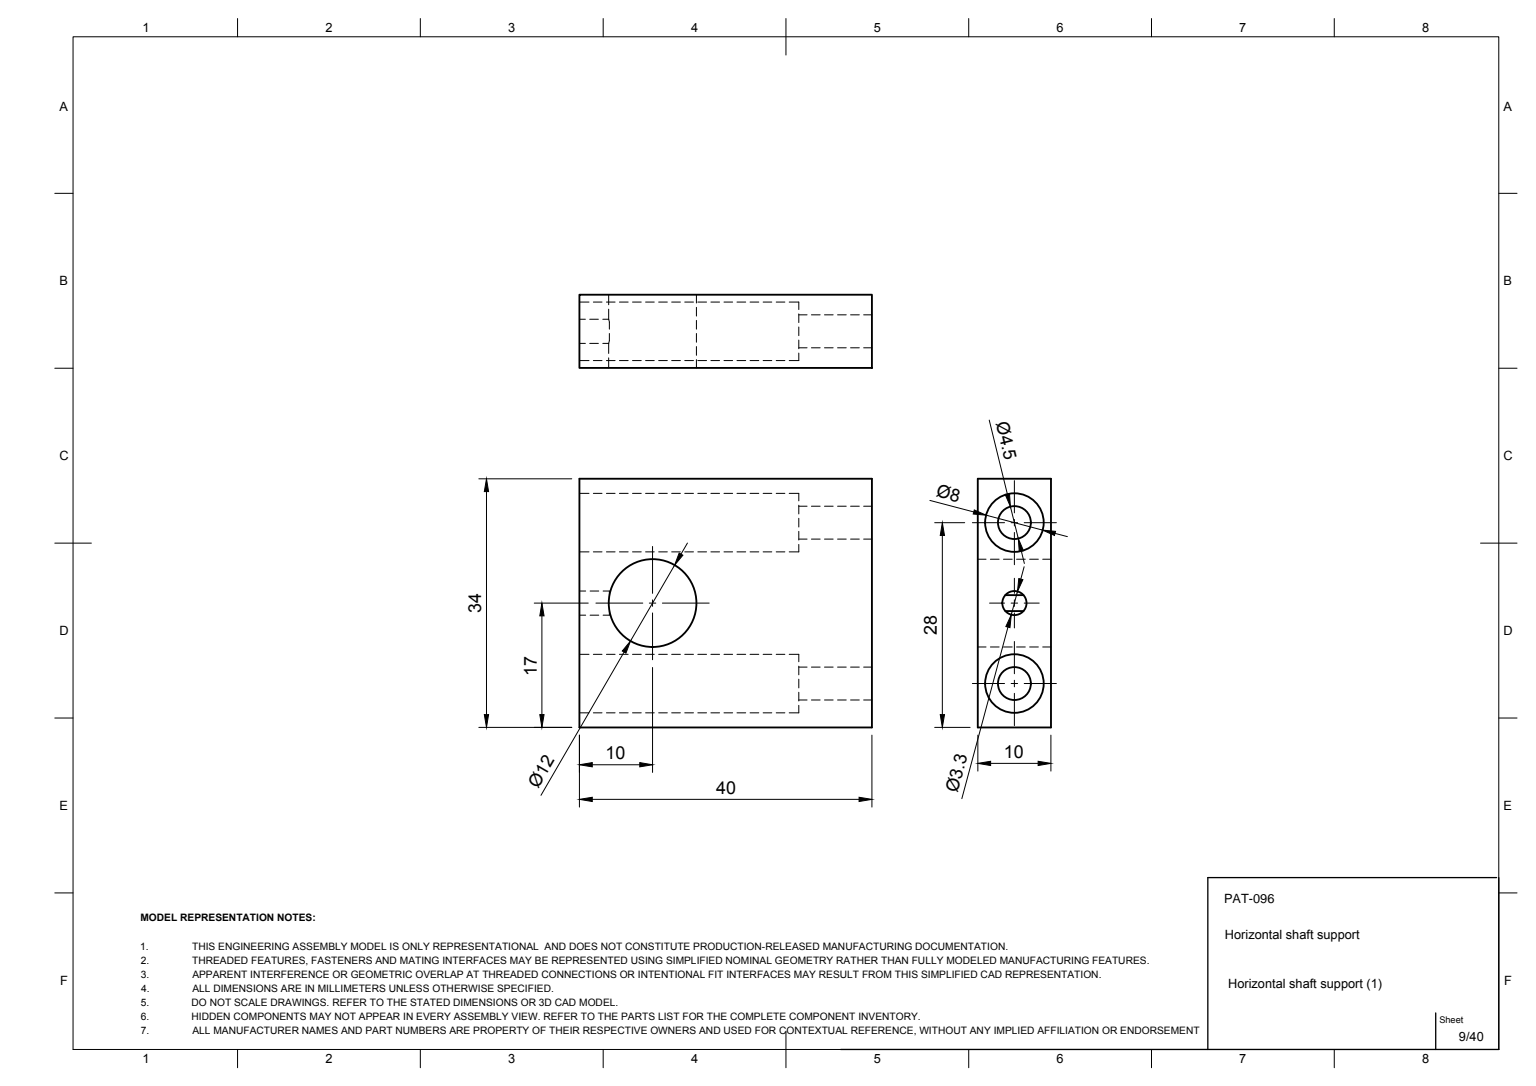
ISO-10303-21;
HEADER;
/* Generated by software containing ST-Developer
 * from STEP Tools, Inc. (www.steptools.com) 
 */

FILE_DESCRIPTION(
/* description */ ('PAT-096'),
/* implementation_level */ '2;1');

FILE_NAME(
/* name */ 'Horizontal shaft support.step',
/* time_stamp */ '2026-10-29T17:03:14-07:00',
/* author */ (''),
/* organization */ (''),
/* preprocessor_version */ 'ST-DEVELOPER v20.2',
/* originating_system */ 'Autodesk Translation Framework v15.17.0.0',
/* authorisation */ '');

FILE_SCHEMA (('AUTOMOTIVE_DESIGN { 1 0 10303 214 3 1 1 }'));
ENDSEC;

DATA;
#10=MECHANICAL_DESIGN_GEOMETRIC_PRESENTATION_REPRESENTATION('',(#416),#10650);
#303=B_SPLINE_CURVE_WITH_KNOTS('',3,(#9562,#9563,#9564,#9565,#9566,#9567),
 .UNSPECIFIED.,.F.,.F.,(4,2,4),(0.635430324955934,0.687528937234029,0.750024497760675),
 .UNSPECIFIED.);
#304=B_SPLINE_CURVE_WITH_KNOTS('',3,(#9571,#9572,#9573,#9574,#9575,#9576),
 .UNSPECIFIED.,.F.,.F.,(4,2,4),(0.250008165920225,0.312503726446871,0.364602338724967),
 .UNSPECIFIED.);
#305=B_SPLINE_CURVE_WITH_KNOTS('',3,(#9577,#9578,#9579,#9580,#9581,#9582),
 .UNSPECIFIED.,.F.,.F.,(4,2,4),(0.135413993115484,0.187512605393579,0.250008165920225),
 .UNSPECIFIED.);
#306=B_SPLINE_CURVE_WITH_KNOTS('',3,(#9583,#9584,#9585,#9586,#9587,#9588),
 .UNSPECIFIED.,.F.,.F.,(4,2,4),(0.750024497760675,0.81252005828732,0.864618670565416),
 .UNSPECIFIED.);
#346=SHAPE_REPRESENTATION_RELATIONSHIP('SRR','None',#10807,#377);
#377=ADVANCED_BREP_SHAPE_REPRESENTATION('',(#454),#10625);
#416=STYLED_ITEM('',(#11064),#454);
#454=MANIFOLD_SOLID_BREP('Body1',#5550);
#532=FACE_BOUND('',#1324,.T.);
#533=FACE_BOUND('',#1327,.T.);
#534=FACE_BOUND('',#1329,.T.);
#535=FACE_BOUND('',#1330,.T.);
#536=FACE_BOUND('',#1331,.T.);
#537=FACE_BOUND('',#1336,.T.);
#538=FACE_BOUND('',#1338,.T.);
#539=FACE_BOUND('',#1340,.T.);
#540=FACE_BOUND('',#1341,.T.);
#667=PLANE('',#6226);
#668=PLANE('',#6227);
#669=PLANE('',#6228);
#670=PLANE('',#6233);
#671=PLANE('',#6237);
#672=PLANE('',#6242);
#673=PLANE('',#6244);
#674=PLANE('',#6252);
#675=PLANE('',#6253);
#676=PLANE('',#6254);
#922=FACE_OUTER_BOUND('',#1317,.T.);
#923=FACE_OUTER_BOUND('',#1318,.T.);
#924=FACE_OUTER_BOUND('',#1319,.T.);
#925=FACE_OUTER_BOUND('',#1320,.T.);
#926=FACE_OUTER_BOUND('',#1321,.T.);
#927=FACE_OUTER_BOUND('',#1322,.T.);
#928=FACE_OUTER_BOUND('',#1323,.T.);
#929=FACE_OUTER_BOUND('',#1325,.T.);
#930=FACE_OUTER_BOUND('',#1326,.T.);
#931=FACE_OUTER_BOUND('',#1328,.T.);
#932=FACE_OUTER_BOUND('',#1332,.T.);
#933=FACE_OUTER_BOUND('',#1333,.T.);
#934=FACE_OUTER_BOUND('',#1334,.T.);
#935=FACE_OUTER_BOUND('',#1335,.T.);
#936=FACE_OUTER_BOUND('',#1337,.T.);
#937=FACE_OUTER_BOUND('',#1339,.T.);
#1317=EDGE_LOOP('',(#4265,#4266,#4267,#4268));
#1318=EDGE_LOOP('',(#4269,#4270,#4271,#4272));
#1319=EDGE_LOOP('',(#4273,#4274));
#1320=EDGE_LOOP('',(#4275,#4276,#4277,#4278,#4279,#4280,#4281,#4282,#4283));
#1321=EDGE_LOOP('',(#4284,#4285));
#1322=EDGE_LOOP('',(#4286,#4287,#4288,#4289));
#1323=EDGE_LOOP('',(#4290));
#1324=EDGE_LOOP('',(#4291));
#1325=EDGE_LOOP('',(#4292,#4293,#4294,#4295));
#1326=EDGE_LOOP('',(#4296));
#1327=EDGE_LOOP('',(#4297));
#1328=EDGE_LOOP('',(#4298,#4299,#4300,#4301));
#1329=EDGE_LOOP('',(#4302));
#1330=EDGE_LOOP('',(#4303));
#1331=EDGE_LOOP('',(#4304));
#1332=EDGE_LOOP('',(#4305,#4306,#4307,#4308));
#1333=EDGE_LOOP('',(#4309,#4310,#4311,#4312));
#1334=EDGE_LOOP('',(#4313,#4314,#4315,#4316,#4317,#4318,#4319,#4320,#4321,
#4322,#4323,#4324));
#1335=EDGE_LOOP('',(#4325,#4326,#4327,#4328));
#1336=EDGE_LOOP('',(#4329));
#1337=EDGE_LOOP('',(#4330,#4331,#4332,#4333));
#1338=EDGE_LOOP('',(#4334));
#1339=EDGE_LOOP('',(#4335,#4336,#4337,#4338));
#1340=EDGE_LOOP('',(#4339));
#1341=EDGE_LOOP('',(#4340));
#1694=LINE('',#9539,#2023);
#1695=LINE('',#9541,#2024);
#1696=LINE('',#9543,#2025);
#1697=LINE('',#9544,#2026);
#1698=LINE('',#9548,#2027);
#1699=LINE('',#9550,#2028);
#1700=LINE('',#9552,#2029);
#1701=LINE('',#9553,#2030);
#1702=LINE('',#9557,#2031);
#1703=LINE('',#9590,#2032);
#1704=LINE('',#9593,#2033);
#1705=LINE('',#9598,#2034);
#1706=LINE('',#9607,#2035);
#1707=LINE('',#9613,#2036);
#1708=LINE('',#9614,#2037);
#1709=LINE('',#9618,#2038);
#1710=LINE('',#9622,#2039);
#1711=LINE('',#9626,#2040);
#1712=LINE('',#9628,#2041);
#1713=LINE('',#9631,#2042);
#1714=LINE('',#9633,#2043);
#2023=VECTOR('',#7388,1.);
#2024=VECTOR('',#7389,1.);
#2025=VECTOR('',#7390,1.);
#2026=VECTOR('',#7391,1.);
#2027=VECTOR('',#7394,1.);
#2028=VECTOR('',#7395,1.);
#2029=VECTOR('',#7396,1.);
#2030=VECTOR('',#7397,1.);
#2031=VECTOR('',#7400,1.);
#2032=VECTOR('',#7407,0.165);
#2033=VECTOR('',#7412,1.);
#2034=VECTOR('',#7417,0.4);
#2035=VECTOR('',#7428,0.4);
#2036=VECTOR('',#7437,1.);
#2037=VECTOR('',#7438,1.);
#2038=VECTOR('',#7443,0.225);
#2039=VECTOR('',#7448,0.225);
#2040=VECTOR('',#7453,0.6);
#2041=VECTOR('',#7454,0.6);
#2042=VECTOR('',#7459,1.);
#2043=VECTOR('',#7462,1.);
#2419=CIRCLE('',#6229,0.165);
#2420=CIRCLE('',#6231,0.165);
#2421=CIRCLE('',#6232,0.165);
#2422=CIRCLE('',#6235,0.4);
#2423=CIRCLE('',#6236,0.4);
#2424=CIRCLE('',#6238,0.225);
#2425=CIRCLE('',#6240,0.4);
#2426=CIRCLE('',#6241,0.4);
#2427=CIRCLE('',#6243,0.225);
#2428=CIRCLE('',#6246,0.225);
#2429=CIRCLE('',#6248,0.225);
#2430=CIRCLE('',#6250,0.6);
#2431=CIRCLE('',#6251,0.6);
#2770=VERTEX_POINT('',#9537);
#2771=VERTEX_POINT('',#9538);
#2772=VERTEX_POINT('',#9540);
#2773=VERTEX_POINT('',#9542);
#2774=VERTEX_POINT('',#9546);
#2775=VERTEX_POINT('',#9547);
#2776=VERTEX_POINT('',#9549);
#2777=VERTEX_POINT('',#9551);
#2778=VERTEX_POINT('',#9555);
#2779=VERTEX_POINT('',#9556);
#2780=VERTEX_POINT('',#9560);
#2781=VERTEX_POINT('',#9561);
#2782=VERTEX_POINT('',#9568);
#2783=VERTEX_POINT('',#9570);
#2784=VERTEX_POINT('',#9589);
#2785=VERTEX_POINT('',#9595);
#2786=VERTEX_POINT('',#9597);
#2787=VERTEX_POINT('',#9601);
#2788=VERTEX_POINT('',#9604);
#2789=VERTEX_POINT('',#9606);
#2790=VERTEX_POINT('',#9610);
#2791=VERTEX_POINT('',#9616);
#2792=VERTEX_POINT('',#9620);
#2793=VERTEX_POINT('',#9624);
#2794=VERTEX_POINT('',#9627);
#3311=EDGE_CURVE('',#2770,#2771,#1694,.T.);
#3312=EDGE_CURVE('',#2771,#2772,#1695,.T.);
#3313=EDGE_CURVE('',#2772,#2773,#1696,.T.);
#3314=EDGE_CURVE('',#2773,#2770,#1697,.T.);
#3315=EDGE_CURVE('',#2774,#2775,#1698,.T.);
#3316=EDGE_CURVE('',#2775,#2776,#1699,.T.);
#3317=EDGE_CURVE('',#2776,#2777,#1700,.T.);
#3318=EDGE_CURVE('',#2777,#2774,#1701,.T.);
#3319=EDGE_CURVE('',#2778,#2779,#1702,.T.);
#3320=EDGE_CURVE('',#2778,#2779,#2419,.T.);
#3321=EDGE_CURVE('',#2780,#2781,#303,.T.);
#3322=EDGE_CURVE('',#2782,#2780,#2420,.T.);
#3323=EDGE_CURVE('',#2783,#2782,#304,.T.);
#3324=EDGE_CURVE('',#2779,#2783,#305,.T.);
#3325=EDGE_CURVE('',#2781,#2778,#306,.T.);
#3326=EDGE_CURVE('',#2781,#2784,#1703,.T.);
#3327=EDGE_CURVE('',#2784,#2784,#2421,.T.);
#3328=EDGE_CURVE('',#2782,#2780,#1704,.T.);
#3329=EDGE_CURVE('',#2785,#2785,#2422,.T.);
#3330=EDGE_CURVE('',#2785,#2786,#1705,.T.);
#3331=EDGE_CURVE('',#2786,#2786,#2423,.T.);
#3332=EDGE_CURVE('',#2787,#2787,#2424,.T.);
#3333=EDGE_CURVE('',#2788,#2788,#2425,.T.);
#3334=EDGE_CURVE('',#2788,#2789,#1706,.T.);
#3335=EDGE_CURVE('',#2789,#2789,#2426,.T.);
#3336=EDGE_CURVE('',#2790,#2790,#2427,.T.);
#3337=EDGE_CURVE('',#2777,#2772,#1707,.T.);
#3338=EDGE_CURVE('',#2773,#2776,#1708,.T.);
#3339=EDGE_CURVE('',#2791,#2791,#2428,.T.);
#3340=EDGE_CURVE('',#2791,#2787,#1709,.T.);
#3341=EDGE_CURVE('',#2792,#2792,#2429,.T.);
#3342=EDGE_CURVE('',#2792,#2790,#1710,.T.);
#3343=EDGE_CURVE('',#2793,#2793,#2430,.T.);
#3344=EDGE_CURVE('',#2793,#2781,#1711,.T.);
#3345=EDGE_CURVE('',#2783,#2794,#1712,.T.);
#3346=EDGE_CURVE('',#2794,#2794,#2431,.T.);
#3347=EDGE_CURVE('',#2770,#2775,#1713,.T.);
#3348=EDGE_CURVE('',#2771,#2774,#1714,.T.);
#4265=ORIENTED_EDGE('',*,*,#3311,.T.);
#4266=ORIENTED_EDGE('',*,*,#3312,.T.);
#4267=ORIENTED_EDGE('',*,*,#3313,.T.);
#4268=ORIENTED_EDGE('',*,*,#3314,.T.);
#4269=ORIENTED_EDGE('',*,*,#3315,.T.);
#4270=ORIENTED_EDGE('',*,*,#3316,.T.);
#4271=ORIENTED_EDGE('',*,*,#3317,.T.);
#4272=ORIENTED_EDGE('',*,*,#3318,.T.);
#4273=ORIENTED_EDGE('',*,*,#3319,.F.);
#4274=ORIENTED_EDGE('',*,*,#3320,.T.);
#4275=ORIENTED_EDGE('',*,*,#3321,.F.);
#4276=ORIENTED_EDGE('',*,*,#3322,.F.);
#4277=ORIENTED_EDGE('',*,*,#3323,.F.);
#4278=ORIENTED_EDGE('',*,*,#3324,.F.);
#4279=ORIENTED_EDGE('',*,*,#3320,.F.);
#4280=ORIENTED_EDGE('',*,*,#3325,.F.);
#4281=ORIENTED_EDGE('',*,*,#3326,.T.);
#4282=ORIENTED_EDGE('',*,*,#3327,.F.);
#4283=ORIENTED_EDGE('',*,*,#3326,.F.);
#4284=ORIENTED_EDGE('',*,*,#3328,.F.);
#4285=ORIENTED_EDGE('',*,*,#3322,.T.);
#4286=ORIENTED_EDGE('',*,*,#3329,.F.);
#4287=ORIENTED_EDGE('',*,*,#3330,.T.);
#4288=ORIENTED_EDGE('',*,*,#3331,.F.);
#4289=ORIENTED_EDGE('',*,*,#3330,.F.);
#4290=ORIENTED_EDGE('',*,*,#3329,.T.);
#4291=ORIENTED_EDGE('',*,*,#3332,.F.);
#4292=ORIENTED_EDGE('',*,*,#3333,.F.);
#4293=ORIENTED_EDGE('',*,*,#3334,.T.);
#4294=ORIENTED_EDGE('',*,*,#3335,.F.);
#4295=ORIENTED_EDGE('',*,*,#3334,.F.);
#4296=ORIENTED_EDGE('',*,*,#3333,.T.);
#4297=ORIENTED_EDGE('',*,*,#3336,.F.);
#4298=ORIENTED_EDGE('',*,*,#3337,.F.);
#4299=ORIENTED_EDGE('',*,*,#3317,.F.);
#4300=ORIENTED_EDGE('',*,*,#3338,.F.);
#4301=ORIENTED_EDGE('',*,*,#3313,.F.);
#4302=ORIENTED_EDGE('',*,*,#3335,.T.);
#4303=ORIENTED_EDGE('',*,*,#3327,.T.);
#4304=ORIENTED_EDGE('',*,*,#3331,.T.);
#4305=ORIENTED_EDGE('',*,*,#3339,.F.);
#4306=ORIENTED_EDGE('',*,*,#3340,.T.);
#4307=ORIENTED_EDGE('',*,*,#3332,.T.);
#4308=ORIENTED_EDGE('',*,*,#3340,.F.);
#4309=ORIENTED_EDGE('',*,*,#3341,.F.);
#4310=ORIENTED_EDGE('',*,*,#3342,.T.);
#4311=ORIENTED_EDGE('',*,*,#3336,.T.);
#4312=ORIENTED_EDGE('',*,*,#3342,.F.);
#4313=ORIENTED_EDGE('',*,*,#3343,.F.);
#4314=ORIENTED_EDGE('',*,*,#3344,.T.);
#4315=ORIENTED_EDGE('',*,*,#3325,.T.);
#4316=ORIENTED_EDGE('',*,*,#3319,.T.);
#4317=ORIENTED_EDGE('',*,*,#3324,.T.);
#4318=ORIENTED_EDGE('',*,*,#3345,.T.);
#4319=ORIENTED_EDGE('',*,*,#3346,.F.);
#4320=ORIENTED_EDGE('',*,*,#3345,.F.);
#4321=ORIENTED_EDGE('',*,*,#3323,.T.);
#4322=ORIENTED_EDGE('',*,*,#3328,.T.);
#4323=ORIENTED_EDGE('',*,*,#3321,.T.);
#4324=ORIENTED_EDGE('',*,*,#3344,.F.);
#4325=ORIENTED_EDGE('',*,*,#3347,.F.);
#4326=ORIENTED_EDGE('',*,*,#3314,.F.);
#4327=ORIENTED_EDGE('',*,*,#3338,.T.);
#4328=ORIENTED_EDGE('',*,*,#3316,.F.);
#4329=ORIENTED_EDGE('',*,*,#3346,.T.);
#4330=ORIENTED_EDGE('',*,*,#3348,.T.);
#4331=ORIENTED_EDGE('',*,*,#3318,.F.);
#4332=ORIENTED_EDGE('',*,*,#3337,.T.);
#4333=ORIENTED_EDGE('',*,*,#3312,.F.);
#4334=ORIENTED_EDGE('',*,*,#3343,.T.);
#4335=ORIENTED_EDGE('',*,*,#3348,.F.);
#4336=ORIENTED_EDGE('',*,*,#3311,.F.);
#4337=ORIENTED_EDGE('',*,*,#3347,.T.);
#4338=ORIENTED_EDGE('',*,*,#3315,.F.);
#4339=ORIENTED_EDGE('',*,*,#3339,.T.);
#4340=ORIENTED_EDGE('',*,*,#3341,.T.);
#5124=CYLINDRICAL_SURFACE('',#6230,0.165);
#5125=CYLINDRICAL_SURFACE('',#6234,0.4);
#5126=CYLINDRICAL_SURFACE('',#6239,0.4);
#5127=CYLINDRICAL_SURFACE('',#6245,0.225);
#5128=CYLINDRICAL_SURFACE('',#6247,0.225);
#5129=CYLINDRICAL_SURFACE('',#6249,0.6);
#5327=ADVANCED_FACE('',(#922),#667,.T.);
#5328=ADVANCED_FACE('',(#923),#668,.T.);
#5329=ADVANCED_FACE('',(#924),#669,.T.);
#5330=ADVANCED_FACE('',(#925),#5124,.F.);
#5331=ADVANCED_FACE('',(#926),#670,.T.);
#5332=ADVANCED_FACE('',(#927),#5125,.F.);
#5333=ADVANCED_FACE('',(#928,#532),#671,.T.);
#5334=ADVANCED_FACE('',(#929),#5126,.F.);
#5335=ADVANCED_FACE('',(#930,#533),#672,.T.);
#5336=ADVANCED_FACE('',(#931,#534,#535,#536),#673,.T.);
#5337=ADVANCED_FACE('',(#932),#5127,.F.);
#5338=ADVANCED_FACE('',(#933),#5128,.F.);
#5339=ADVANCED_FACE('',(#934),#5129,.F.);
#5340=ADVANCED_FACE('',(#935,#537),#674,.T.);
#5341=ADVANCED_FACE('',(#936,#538),#675,.T.);
#5342=ADVANCED_FACE('',(#937,#539,#540),#676,.F.);
#5550=CLOSED_SHELL('',(#5327,#5328,#5329,#5330,#5331,#5332,#5333,#5334,
#5335,#5336,#5337,#5338,#5339,#5340,#5341,#5342));
#6225=AXIS2_PLACEMENT_3D('',#9535,#7384,#7385);
#6226=AXIS2_PLACEMENT_3D('',#9536,#7386,#7387);
#6227=AXIS2_PLACEMENT_3D('',#9545,#7392,#7393);
#6228=AXIS2_PLACEMENT_3D('',#9554,#7398,#7399);
#6229=AXIS2_PLACEMENT_3D('',#9558,#7401,#7402);
#6230=AXIS2_PLACEMENT_3D('',#9559,#7403,#7404);
#6231=AXIS2_PLACEMENT_3D('',#9569,#7405,#7406);
#6232=AXIS2_PLACEMENT_3D('',#9591,#7408,#7409);
#6233=AXIS2_PLACEMENT_3D('',#9592,#7410,#7411);
#6234=AXIS2_PLACEMENT_3D('',#9594,#7413,#7414);
#6235=AXIS2_PLACEMENT_3D('',#9596,#7415,#7416);
#6236=AXIS2_PLACEMENT_3D('',#9599,#7418,#7419);
#6237=AXIS2_PLACEMENT_3D('',#9600,#7420,#7421);
#6238=AXIS2_PLACEMENT_3D('',#9602,#7422,#7423);
#6239=AXIS2_PLACEMENT_3D('',#9603,#7424,#7425);
#6240=AXIS2_PLACEMENT_3D('',#9605,#7426,#7427);
#6241=AXIS2_PLACEMENT_3D('',#9608,#7429,#7430);
#6242=AXIS2_PLACEMENT_3D('',#9609,#7431,#7432);
#6243=AXIS2_PLACEMENT_3D('',#9611,#7433,#7434);
#6244=AXIS2_PLACEMENT_3D('',#9612,#7435,#7436);
#6245=AXIS2_PLACEMENT_3D('',#9615,#7439,#7440);
#6246=AXIS2_PLACEMENT_3D('',#9617,#7441,#7442);
#6247=AXIS2_PLACEMENT_3D('',#9619,#7444,#7445);
#6248=AXIS2_PLACEMENT_3D('',#9621,#7446,#7447);
#6249=AXIS2_PLACEMENT_3D('',#9623,#7449,#7450);
#6250=AXIS2_PLACEMENT_3D('',#9625,#7451,#7452);
#6251=AXIS2_PLACEMENT_3D('',#9629,#7455,#7456);
#6252=AXIS2_PLACEMENT_3D('',#9630,#7457,#7458);
#6253=AXIS2_PLACEMENT_3D('',#9632,#7460,#7461);
#6254=AXIS2_PLACEMENT_3D('',#9634,#7463,#7464);
#7384=DIRECTION('axis',(0.,0.,1.));
#7385=DIRECTION('refdir',(1.,0.,0.));
#7386=DIRECTION('center_axis',(0.,1.,0.));
#7387=DIRECTION('ref_axis',(0.,0.,1.));
#7388=DIRECTION('',(-1.,0.,0.));
#7389=DIRECTION('',(0.,0.,1.));
#7390=DIRECTION('',(1.,0.,0.));
#7391=DIRECTION('',(0.,0.,-1.));
#7392=DIRECTION('center_axis',(0.,-1.,0.));
#7393=DIRECTION('ref_axis',(0.,0.,-1.));
#7394=DIRECTION('',(1.,0.,0.));
#7395=DIRECTION('',(0.,0.,1.));
#7396=DIRECTION('',(-1.,0.,0.));
#7397=DIRECTION('',(0.,0.,-1.));
#7398=DIRECTION('center_axis',(0.,0.,1.));
#7399=DIRECTION('ref_axis',(1.,0.,0.));
#7400=DIRECTION('',(1.,0.,0.));
#7401=DIRECTION('center_axis',(0.,0.,1.));
#7402=DIRECTION('ref_axis',(1.,0.,0.));
#7403=DIRECTION('center_axis',(0.,0.,1.));
#7404=DIRECTION('ref_axis',(1.,0.,0.));
#7405=DIRECTION('center_axis',(0.,0.,1.));
#7406=DIRECTION('ref_axis',(1.,0.,0.));
#7407=DIRECTION('',(0.,0.,1.));
#7408=DIRECTION('center_axis',(0.,0.,-1.));
#7409=DIRECTION('ref_axis',(1.,0.,0.));
#7410=DIRECTION('center_axis',(0.,0.,1.));
#7411=DIRECTION('ref_axis',(1.,0.,0.));
#7412=DIRECTION('',(-1.,0.,0.));
#7413=DIRECTION('center_axis',(0.,0.,1.));
#7414=DIRECTION('ref_axis',(1.,0.,0.));
#7415=DIRECTION('center_axis',(0.,0.,1.));
#7416=DIRECTION('ref_axis',(1.,0.,0.));
#7417=DIRECTION('',(0.,0.,1.));
#7418=DIRECTION('center_axis',(0.,0.,-1.));
#7419=DIRECTION('ref_axis',(1.,0.,0.));
#7420=DIRECTION('center_axis',(0.,0.,1.));
#7421=DIRECTION('ref_axis',(1.,0.,0.));
#7422=DIRECTION('center_axis',(0.,0.,1.));
#7423=DIRECTION('ref_axis',(1.,0.,0.));
#7424=DIRECTION('center_axis',(0.,0.,1.));
#7425=DIRECTION('ref_axis',(1.,0.,0.));
#7426=DIRECTION('center_axis',(0.,0.,1.));
#7427=DIRECTION('ref_axis',(1.,0.,0.));
#7428=DIRECTION('',(0.,0.,1.));
#7429=DIRECTION('center_axis',(0.,0.,-1.));
#7430=DIRECTION('ref_axis',(1.,0.,0.));
#7431=DIRECTION('center_axis',(0.,0.,1.));
#7432=DIRECTION('ref_axis',(1.,0.,0.));
#7433=DIRECTION('center_axis',(0.,0.,1.));
#7434=DIRECTION('ref_axis',(1.,0.,0.));
#7435=DIRECTION('center_axis',(0.,0.,1.));
#7436=DIRECTION('ref_axis',(1.,0.,0.));
#7437=DIRECTION('',(0.,1.,0.));
#7438=DIRECTION('',(0.,-1.,0.));
#7439=DIRECTION('center_axis',(0.,0.,1.));
#7440=DIRECTION('ref_axis',(1.,0.,0.));
#7441=DIRECTION('center_axis',(0.,0.,1.));
#7442=DIRECTION('ref_axis',(1.,0.,0.));
#7443=DIRECTION('',(0.,0.,1.));
#7444=DIRECTION('center_axis',(0.,0.,1.));
#7445=DIRECTION('ref_axis',(1.,0.,0.));
#7446=DIRECTION('center_axis',(0.,0.,1.));
#7447=DIRECTION('ref_axis',(1.,0.,0.));
#7448=DIRECTION('',(0.,0.,1.));
#7449=DIRECTION('center_axis',(1.,0.,0.));
#7450=DIRECTION('ref_axis',(0.,0.,-1.));
#7451=DIRECTION('center_axis',(1.,0.,0.));
#7452=DIRECTION('ref_axis',(0.,0.,-1.));
#7453=DIRECTION('',(1.,0.,0.));
#7454=DIRECTION('',(1.,0.,0.));
#7455=DIRECTION('center_axis',(-1.,0.,0.));
#7456=DIRECTION('ref_axis',(0.,0.,-1.));
#7457=DIRECTION('center_axis',(1.,0.,0.));
#7458=DIRECTION('ref_axis',(0.,1.,0.));
#7459=DIRECTION('',(0.,-1.,0.));
#7460=DIRECTION('center_axis',(-1.,0.,0.));
#7461=DIRECTION('ref_axis',(0.,-1.,0.));
#7462=DIRECTION('',(0.,-1.,0.));
#7463=DIRECTION('center_axis',(0.,0.,1.));
#7464=DIRECTION('ref_axis',(1.,0.,0.));
#9535=CARTESIAN_POINT('',(0.,0.,0.));
#9536=CARTESIAN_POINT('Origin',(6.,3.7,1.));
#9537=CARTESIAN_POINT('',(6.,3.7,1.));
#9538=CARTESIAN_POINT('',(5.,3.7,1.));
#9539=CARTESIAN_POINT('',(6.,3.7,1.));
#9540=CARTESIAN_POINT('',(5.,3.7,5.));
#9541=CARTESIAN_POINT('',(5.,3.7,1.));
#9542=CARTESIAN_POINT('',(6.,3.7,5.));
#9543=CARTESIAN_POINT('',(6.,3.7,5.));
#9544=CARTESIAN_POINT('',(6.,3.7,1.));
#9545=CARTESIAN_POINT('Origin',(5.,0.3,1.));
#9546=CARTESIAN_POINT('',(5.,0.3,1.));
#9547=CARTESIAN_POINT('',(6.,0.3,1.));
#9548=CARTESIAN_POINT('',(5.,0.3,1.));
#9549=CARTESIAN_POINT('',(6.,0.3,5.));
#9550=CARTESIAN_POINT('',(6.,0.3,1.));
#9551=CARTESIAN_POINT('',(5.,0.3,5.));
#9552=CARTESIAN_POINT('',(5.,0.3,5.));
#9553=CARTESIAN_POINT('',(5.,0.3,1.));
#9554=CARTESIAN_POINT('Origin',(5.5,2.,4.59));
#9555=CARTESIAN_POINT('',(5.3762058159686,1.89091287885364,4.59));
#9556=CARTESIAN_POINT('',(5.6237941840314,1.89091287885364,4.59));
#9557=CARTESIAN_POINT('',(4.9,1.89091287885364,4.59));
#9558=CARTESIAN_POINT('Origin',(5.5,2.,4.59));
#9559=CARTESIAN_POINT('Origin',(5.5,2.,4.59));
#9560=CARTESIAN_POINT('',(5.3762058159686,2.10908712114636,4.59));
#9561=CARTESIAN_POINT('',(5.335,2.,4.6));
#9562=CARTESIAN_POINT('Ctrl Pts',(5.3762058159686,2.10908712114636,4.59));
#9563=CARTESIAN_POINT('Ctrl Pts',(5.36460086481047,2.09591759715261,4.59243495840567));
#9564=CARTESIAN_POINT('Ctrl Pts',(5.35465435634175,2.08022344943772,4.59485638705045));
#9565=CARTESIAN_POINT('Ctrl Pts',(5.33918513536598,2.04298016596019,4.59880705606552));
#9566=CARTESIAN_POINT('Ctrl Pts',(5.335,2.02083185350888,4.6));
#9567=CARTESIAN_POINT('Ctrl Pts',(5.335,2.,4.6));
#9568=CARTESIAN_POINT('',(5.6237941840314,2.10908712114636,4.59));
#9569=CARTESIAN_POINT('Origin',(5.5,2.,4.59));
#9570=CARTESIAN_POINT('',(5.665,2.,4.6));
#9571=CARTESIAN_POINT('Ctrl Pts',(5.665,2.,4.6));
#9572=CARTESIAN_POINT('Ctrl Pts',(5.665,2.02083185350888,4.6));
#9573=CARTESIAN_POINT('Ctrl Pts',(5.66081486463402,2.04298016596019,4.59880705606552));
#9574=CARTESIAN_POINT('Ctrl Pts',(5.64534564365825,2.08022344943772,4.59485638705045));
#9575=CARTESIAN_POINT('Ctrl Pts',(5.63539913518953,2.09591759715261,4.59243495840567));
#9576=CARTESIAN_POINT('Ctrl Pts',(5.6237941840314,2.10908712114636,4.59));
#9577=CARTESIAN_POINT('Ctrl Pts',(5.6237941840314,1.89091287885364,4.59));
#9578=CARTESIAN_POINT('Ctrl Pts',(5.63539913518953,1.90408240284739,4.59243495840567));
#9579=CARTESIAN_POINT('Ctrl Pts',(5.64534564365825,1.91977655056228,4.59485638705045));
#9580=CARTESIAN_POINT('Ctrl Pts',(5.66081486463402,1.95701983403981,4.59880705606552));
#9581=CARTESIAN_POINT('Ctrl Pts',(5.665,1.97916814649112,4.6));
#9582=CARTESIAN_POINT('Ctrl Pts',(5.665,2.,4.6));
#9583=CARTESIAN_POINT('Ctrl Pts',(5.335,2.,4.6));
#9584=CARTESIAN_POINT('Ctrl Pts',(5.335,1.97916814649112,4.6));
#9585=CARTESIAN_POINT('Ctrl Pts',(5.33918513536598,1.95701983403981,4.59880705606552));
#9586=CARTESIAN_POINT('Ctrl Pts',(5.35465435634175,1.91977655056228,4.59485638705045));
#9587=CARTESIAN_POINT('Ctrl Pts',(5.36460086481047,1.90408240284739,4.59243495840567));
#9588=CARTESIAN_POINT('Ctrl Pts',(5.3762058159686,1.89091287885364,4.59));
#9589=CARTESIAN_POINT('',(5.335,2.,5.));
#9590=CARTESIAN_POINT('',(5.335,2.,4.59));
#9591=CARTESIAN_POINT('Origin',(5.5,2.,5.));
#9592=CARTESIAN_POINT('Origin',(5.5,2.,4.59));
#9593=CARTESIAN_POINT('',(4.9,2.10908712114636,4.59));
#9594=CARTESIAN_POINT('Origin',(5.5,0.9,2.));
#9595=CARTESIAN_POINT('',(5.1,0.9,2.));
#9596=CARTESIAN_POINT('Origin',(5.5,0.9,2.));
#9597=CARTESIAN_POINT('',(5.1,0.9,5.));
#9598=CARTESIAN_POINT('',(5.1,0.9,2.));
#9599=CARTESIAN_POINT('Origin',(5.5,0.9,5.));
#9600=CARTESIAN_POINT('Origin',(5.5,0.9,2.));
#9601=CARTESIAN_POINT('',(5.275,0.9,2.));
#9602=CARTESIAN_POINT('Origin',(5.5,0.9,2.));
#9603=CARTESIAN_POINT('Origin',(5.5,3.1,2.));
#9604=CARTESIAN_POINT('',(5.1,3.1,2.));
#9605=CARTESIAN_POINT('Origin',(5.5,3.1,2.));
#9606=CARTESIAN_POINT('',(5.1,3.1,5.));
#9607=CARTESIAN_POINT('',(5.1,3.1,2.));
#9608=CARTESIAN_POINT('Origin',(5.5,3.1,5.));
#9609=CARTESIAN_POINT('Origin',(5.5,3.1,2.));
#9610=CARTESIAN_POINT('',(5.275,3.1,2.));
#9611=CARTESIAN_POINT('Origin',(5.5,3.1,2.));
#9612=CARTESIAN_POINT('Origin',(5.5,2.,5.));
#9613=CARTESIAN_POINT('',(5.,3.5,5.));
#9614=CARTESIAN_POINT('',(6.,0.5,5.));
#9615=CARTESIAN_POINT('Origin',(5.5,0.9,0.9));
#9616=CARTESIAN_POINT('',(5.275,0.9,1.));
#9617=CARTESIAN_POINT('Origin',(5.5,0.9,1.));
#9618=CARTESIAN_POINT('',(5.275,0.9,0.9));
#9619=CARTESIAN_POINT('Origin',(5.5,3.1,0.9));
#9620=CARTESIAN_POINT('',(5.275,3.1,1.));
#9621=CARTESIAN_POINT('Origin',(5.5,3.1,1.));
#9622=CARTESIAN_POINT('',(5.275,3.1,0.9));
#9623=CARTESIAN_POINT('Origin',(4.9,2.,4.));
#9624=CARTESIAN_POINT('',(5.,2.,4.6));
#9625=CARTESIAN_POINT('Origin',(5.,2.,4.));
#9626=CARTESIAN_POINT('',(4.9,2.,4.6));
#9627=CARTESIAN_POINT('',(6.,2.,4.6));
#9628=CARTESIAN_POINT('',(4.9,2.,4.6));
#9629=CARTESIAN_POINT('Origin',(6.,2.,4.));
#9630=CARTESIAN_POINT('Origin',(6.,0.5,1.));
#9631=CARTESIAN_POINT('',(6.,0.5,1.));
#9632=CARTESIAN_POINT('Origin',(5.,3.5,1.));
#9633=CARTESIAN_POINT('',(5.,3.5,1.));
#9634=CARTESIAN_POINT('Origin',(5.5,2.,1.));
#10586=UNCERTAINTY_MEASURE_WITH_UNIT(LENGTH_MEASURE(0.001),#10651,
'DISTANCE_ACCURACY_VALUE',
'Maximum model space distance between geometric entities at asserted c
onnectivities');
#10611=UNCERTAINTY_MEASURE_WITH_UNIT(LENGTH_MEASURE(0.001),#10651,
'DISTANCE_ACCURACY_VALUE',
'Maximum model space distance between geometric entities at asserted c
onnectivities');
#10625=(
GEOMETRIC_REPRESENTATION_CONTEXT(3)
GLOBAL_UNCERTAINTY_ASSIGNED_CONTEXT((#10586))
GLOBAL_UNIT_ASSIGNED_CONTEXT((#10651,#10653,#10654))
REPRESENTATION_CONTEXT('','3D')
);
#10650=(
GEOMETRIC_REPRESENTATION_CONTEXT(3)
GLOBAL_UNCERTAINTY_ASSIGNED_CONTEXT((#10611))
GLOBAL_UNIT_ASSIGNED_CONTEXT((#10651,#10653,#10654))
REPRESENTATION_CONTEXT('','3D')
);
#10651=(
LENGTH_UNIT()
NAMED_UNIT(*)
SI_UNIT(.CENTI.,.METRE.)
);
#10653=(
NAMED_UNIT(*)
PLANE_ANGLE_UNIT()
SI_UNIT($,.RADIAN.)
);
#10654=(
NAMED_UNIT(*)
SI_UNIT($,.STERADIAN.)
SOLID_ANGLE_UNIT()
);
#10668=SHAPE_DEFINITION_REPRESENTATION(#10711,#10807);
#10711=PRODUCT_DEFINITION_SHAPE('',$,#10846);
#10807=SHAPE_REPRESENTATION('',(#6225),#10625);
#10832=PRODUCT_DEFINITION_CONTEXT('part definition',#10948,'design');
#10846=PRODUCT_DEFINITION('Horizontal shaft support',
'Horizontal shaft support',#10884,#10832);
#10884=PRODUCT_DEFINITION_FORMATION('',$,#10963);
#10948=APPLICATION_CONTEXT(
'Core Data for Automotive Mechanical Design Process');
#10949=PRODUCT_CONTEXT('part definition',#10948,'mechanical');
#10963=PRODUCT('Horizontal shaft support','Horizontal shaft support',
'Horizontal shaft support',(#10949));
#11058=COLOUR_RGB('Grey',0.48,0.52,0.57);
#11059=FILL_AREA_STYLE_COLOUR('',#11058);
#11060=FILL_AREA_STYLE('',(#11059));
#11061=SURFACE_STYLE_FILL_AREA(#11060);
#11062=SURFACE_SIDE_STYLE('',(#11061));
#11063=SURFACE_STYLE_USAGE(.BOTH.,#11062);
#11064=PRESENTATION_STYLE_ASSIGNMENT((#11063));
ENDSEC;
END-ISO-10303-21;
